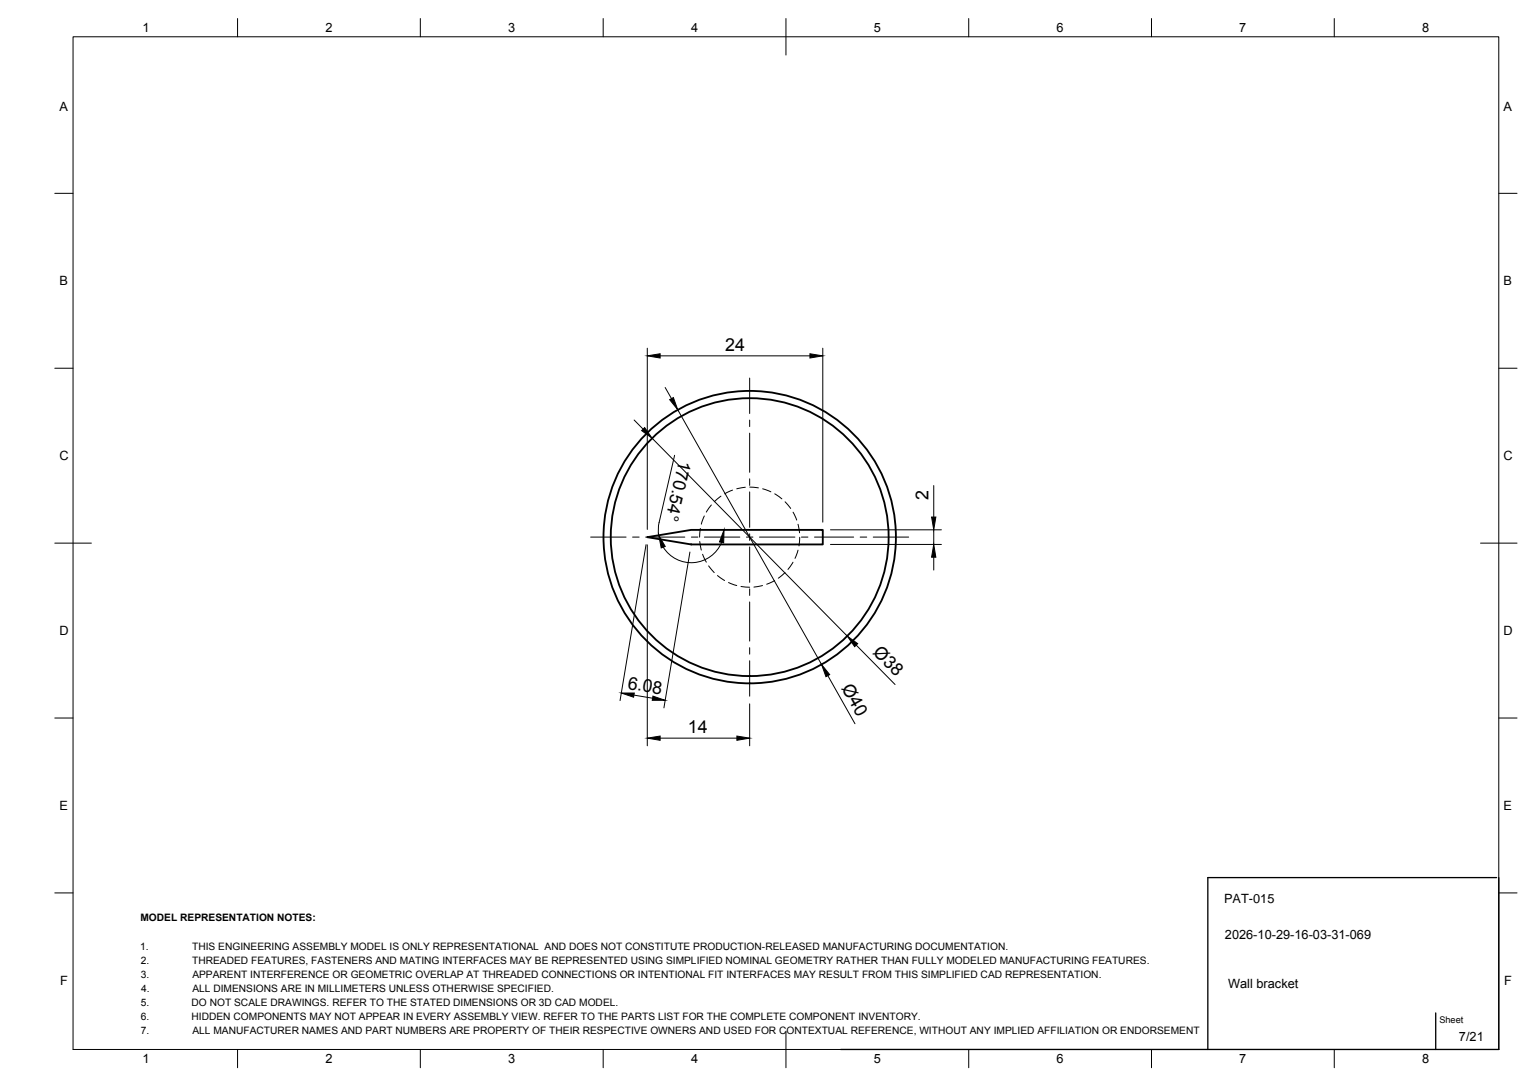
ISO-10303-21;
HEADER;
/* Generated by software containing ST-Developer
 * from STEP Tools, Inc. (www.steptools.com) 
 */

FILE_DESCRIPTION(
/* description */ ('PAT-015'),
/* implementation_level */ '2;1');

FILE_NAME(
/* name */ 'Wall bracket.step',
/* time_stamp */ '2026-10-29T16:03:43-07:00',
/* author */ (''),
/* organization */ (''),
/* preprocessor_version */ 'ST-DEVELOPER v20.2',
/* originating_system */ 'Autodesk Translation Framework v15.17.0.0',
/* authorisation */ '');

FILE_SCHEMA (('AUTOMOTIVE_DESIGN { 1 0 10303 214 3 1 1 }'));
ENDSEC;

DATA;
#10=MECHANICAL_DESIGN_GEOMETRIC_PRESENTATION_REPRESENTATION('',(#236),#10266);
#188=SHAPE_REPRESENTATION_RELATIONSHIP('SRR','None',#10359,#211);
#211=ADVANCED_BREP_SHAPE_REPRESENTATION('',(#261),#10247);
#236=STYLED_ITEM('',(#10526),#261);
#261=MANIFOLD_SOLID_BREP('Body1',#4695);
#346=FACE_BOUND('',#1016,.T.);
#347=FACE_BOUND('',#1017,.T.);
#348=FACE_BOUND('',#1019,.T.);
#349=FACE_BOUND('',#1020,.T.);
#350=FACE_BOUND('',#1024,.T.);
#351=FACE_BOUND('',#1025,.T.);
#352=FACE_BOUND('',#1026,.T.);
#353=FACE_BOUND('',#1027,.T.);
#354=FACE_BOUND('',#1033,.T.);
#355=FACE_BOUND('',#1034,.T.);
#356=FACE_BOUND('',#1035,.T.);
#357=FACE_BOUND('',#1037,.T.);
#358=FACE_BOUND('',#1038,.T.);
#359=FACE_BOUND('',#1039,.T.);
#467=PLANE('',#5185);
#468=PLANE('',#5186);
#469=PLANE('',#5187);
#470=PLANE('',#5188);
#471=PLANE('',#5189);
#472=PLANE('',#5193);
#473=PLANE('',#5194);
#474=PLANE('',#5195);
#475=PLANE('',#5196);
#476=PLANE('',#5197);
#672=FACE_OUTER_BOUND('',#1009,.T.);
#673=FACE_OUTER_BOUND('',#1010,.T.);
#674=FACE_OUTER_BOUND('',#1011,.T.);
#675=FACE_OUTER_BOUND('',#1012,.T.);
#676=FACE_OUTER_BOUND('',#1013,.T.);
#677=FACE_OUTER_BOUND('',#1014,.T.);
#678=FACE_OUTER_BOUND('',#1015,.T.);
#679=FACE_OUTER_BOUND('',#1018,.T.);
#680=FACE_OUTER_BOUND('',#1021,.T.);
#681=FACE_OUTER_BOUND('',#1022,.T.);
#682=FACE_OUTER_BOUND('',#1023,.T.);
#683=FACE_OUTER_BOUND('',#1028,.T.);
#684=FACE_OUTER_BOUND('',#1029,.T.);
#685=FACE_OUTER_BOUND('',#1030,.T.);
#686=FACE_OUTER_BOUND('',#1031,.T.);
#687=FACE_OUTER_BOUND('',#1032,.T.);
#688=FACE_OUTER_BOUND('',#1036,.T.);
#1009=EDGE_LOOP('',(#3553,#3554,#3555,#3556));
#1010=EDGE_LOOP('',(#3557,#3558,#3559,#3560));
#1011=EDGE_LOOP('',(#3561,#3562,#3563,#3564));
#1012=EDGE_LOOP('',(#3565,#3566,#3567,#3568));
#1013=EDGE_LOOP('',(#3569,#3570,#3571,#3572));
#1014=EDGE_LOOP('',(#3573,#3574,#3575,#3576));
#1015=EDGE_LOOP('',(#3577,#3578,#3579,#3580));
#1016=EDGE_LOOP('',(#3581));
#1017=EDGE_LOOP('',(#3582));
#1018=EDGE_LOOP('',(#3583,#3584,#3585,#3586));
#1019=EDGE_LOOP('',(#3587));
#1020=EDGE_LOOP('',(#3588));
#1021=EDGE_LOOP('',(#3589,#3590,#3591,#3592));
#1022=EDGE_LOOP('',(#3593,#3594,#3595,#3596));
#1023=EDGE_LOOP('',(#3597,#3598,#3599,#3600));
#1024=EDGE_LOOP('',(#3601));
#1025=EDGE_LOOP('',(#3602));
#1026=EDGE_LOOP('',(#3603));
#1027=EDGE_LOOP('',(#3604));
#1028=EDGE_LOOP('',(#3605,#3606,#3607,#3608));
#1029=EDGE_LOOP('',(#3609,#3610,#3611,#3612,#3613,#3614,#3615,#3616));
#1030=EDGE_LOOP('',(#3617,#3618,#3619,#3620));
#1031=EDGE_LOOP('',(#3621,#3622,#3623,#3624,#3625,#3626,#3627,#3628));
#1032=EDGE_LOOP('',(#3629,#3630,#3631,#3632));
#1033=EDGE_LOOP('',(#3633));
#1034=EDGE_LOOP('',(#3634));
#1035=EDGE_LOOP('',(#3635));
#1036=EDGE_LOOP('',(#3636,#3637,#3638,#3639));
#1037=EDGE_LOOP('',(#3640));
#1038=EDGE_LOOP('',(#3641));
#1039=EDGE_LOOP('',(#3642));
#1405=LINE('',#8522,#1685);
#1406=LINE('',#8528,#1686);
#1407=LINE('',#8534,#1687);
#1408=LINE('',#8540,#1688);
#1409=LINE('',#8546,#1689);
#1410=LINE('',#8552,#1690);
#1411=LINE('',#8557,#1691);
#1412=LINE('',#8559,#1692);
#1413=LINE('',#8561,#1693);
#1414=LINE('',#8562,#1694);
#1415=LINE('',#8566,#1695);
#1416=LINE('',#8568,#1696);
#1417=LINE('',#8570,#1697);
#1418=LINE('',#8571,#1698);
#1419=LINE('',#8574,#1699);
#1420=LINE('',#8576,#1700);
#1421=LINE('',#8577,#1701);
#1422=LINE('',#8580,#1702);
#1423=LINE('',#8582,#1703);
#1424=LINE('',#8583,#1704);
#1425=LINE('',#8585,#1705);
#1426=LINE('',#8586,#1706);
#1427=LINE('',#8591,#1707);
#1428=LINE('',#8595,#1708);
#1429=LINE('',#8597,#1709);
#1430=LINE('',#8598,#1710);
#1431=LINE('',#8601,#1711);
#1432=LINE('',#8603,#1712);
#1433=LINE('',#8604,#1713);
#1434=LINE('',#8606,#1714);
#1435=LINE('',#8607,#1715);
#1685=VECTOR('',#6036,0.225);
#1686=VECTOR('',#6043,0.225);
#1687=VECTOR('',#6050,0.33);
#1688=VECTOR('',#6057,0.33);
#1689=VECTOR('',#6064,0.33);
#1690=VECTOR('',#6071,0.33);
#1691=VECTOR('',#6076,1.);
#1692=VECTOR('',#6077,1.);
#1693=VECTOR('',#6078,1.);
#1694=VECTOR('',#6079,1.);
#1695=VECTOR('',#6082,1.);
#1696=VECTOR('',#6083,1.);
#1697=VECTOR('',#6084,1.);
#1698=VECTOR('',#6085,1.);
#1699=VECTOR('',#6088,1.);
#1700=VECTOR('',#6089,1.);
#1701=VECTOR('',#6090,1.);
#1702=VECTOR('',#6093,1.);
#1703=VECTOR('',#6094,1.);
#1704=VECTOR('',#6095,1.);
#1705=VECTOR('',#6098,1.);
#1706=VECTOR('',#6099,1.);
#1707=VECTOR('',#6104,3.4);
#1708=VECTOR('',#6109,1.);
#1709=VECTOR('',#6110,1.);
#1710=VECTOR('',#6111,1.);
#1711=VECTOR('',#6114,1.);
#1712=VECTOR('',#6115,1.);
#1713=VECTOR('',#6116,1.);
#1714=VECTOR('',#6119,1.);
#1715=VECTOR('',#6120,1.);
#1959=CIRCLE('',#5168,0.225);
#1960=CIRCLE('',#5169,0.225);
#1961=CIRCLE('',#5171,0.225);
#1962=CIRCLE('',#5172,0.225);
#1963=CIRCLE('',#5174,0.33);
#1964=CIRCLE('',#5175,0.33);
#1965=CIRCLE('',#5177,0.33);
#1966=CIRCLE('',#5178,0.33);
#1967=CIRCLE('',#5180,0.33);
#1968=CIRCLE('',#5181,0.33);
#1969=CIRCLE('',#5183,0.33);
#1970=CIRCLE('',#5184,0.33);
#1971=CIRCLE('',#5191,3.4);
#1972=CIRCLE('',#5192,3.4);
#2265=VERTEX_POINT('',#8519);
#2266=VERTEX_POINT('',#8521);
#2267=VERTEX_POINT('',#8525);
#2268=VERTEX_POINT('',#8527);
#2269=VERTEX_POINT('',#8531);
#2270=VERTEX_POINT('',#8533);
#2271=VERTEX_POINT('',#8537);
#2272=VERTEX_POINT('',#8539);
#2273=VERTEX_POINT('',#8543);
#2274=VERTEX_POINT('',#8545);
#2275=VERTEX_POINT('',#8549);
#2276=VERTEX_POINT('',#8551);
#2277=VERTEX_POINT('',#8555);
#2278=VERTEX_POINT('',#8556);
#2279=VERTEX_POINT('',#8558);
#2280=VERTEX_POINT('',#8560);
#2281=VERTEX_POINT('',#8564);
#2282=VERTEX_POINT('',#8565);
#2283=VERTEX_POINT('',#8567);
#2284=VERTEX_POINT('',#8569);
#2285=VERTEX_POINT('',#8573);
#2286=VERTEX_POINT('',#8575);
#2287=VERTEX_POINT('',#8579);
#2288=VERTEX_POINT('',#8581);
#2289=VERTEX_POINT('',#8588);
#2290=VERTEX_POINT('',#8590);
#2291=VERTEX_POINT('',#8594);
#2292=VERTEX_POINT('',#8596);
#2293=VERTEX_POINT('',#8600);
#2294=VERTEX_POINT('',#8602);
#2732=EDGE_CURVE('',#2265,#2265,#1959,.T.);
#2733=EDGE_CURVE('',#2265,#2266,#1405,.T.);
#2734=EDGE_CURVE('',#2266,#2266,#1960,.T.);
#2735=EDGE_CURVE('',#2267,#2267,#1961,.T.);
#2736=EDGE_CURVE('',#2267,#2268,#1406,.T.);
#2737=EDGE_CURVE('',#2268,#2268,#1962,.T.);
#2738=EDGE_CURVE('',#2269,#2269,#1963,.T.);
#2739=EDGE_CURVE('',#2269,#2270,#1407,.T.);
#2740=EDGE_CURVE('',#2270,#2270,#1964,.T.);
#2741=EDGE_CURVE('',#2271,#2271,#1965,.T.);
#2742=EDGE_CURVE('',#2271,#2272,#1408,.T.);
#2743=EDGE_CURVE('',#2272,#2272,#1966,.T.);
#2744=EDGE_CURVE('',#2273,#2273,#1967,.T.);
#2745=EDGE_CURVE('',#2273,#2274,#1409,.T.);
#2746=EDGE_CURVE('',#2274,#2274,#1968,.T.);
#2747=EDGE_CURVE('',#2275,#2275,#1969,.T.);
#2748=EDGE_CURVE('',#2275,#2276,#1410,.T.);
#2749=EDGE_CURVE('',#2276,#2276,#1970,.T.);
#2750=EDGE_CURVE('',#2277,#2278,#1411,.T.);
#2751=EDGE_CURVE('',#2278,#2279,#1412,.T.);
#2752=EDGE_CURVE('',#2279,#2280,#1413,.T.);
#2753=EDGE_CURVE('',#2280,#2277,#1414,.T.);
#2754=EDGE_CURVE('',#2281,#2282,#1415,.T.);
#2755=EDGE_CURVE('',#2281,#2283,#1416,.T.);
#2756=EDGE_CURVE('',#2283,#2284,#1417,.T.);
#2757=EDGE_CURVE('',#2284,#2282,#1418,.T.);
#2758=EDGE_CURVE('',#2279,#2285,#1419,.T.);
#2759=EDGE_CURVE('',#2286,#2285,#1420,.T.);
#2760=EDGE_CURVE('',#2280,#2286,#1421,.T.);
#2761=EDGE_CURVE('',#2283,#2287,#1422,.T.);
#2762=EDGE_CURVE('',#2288,#2287,#1423,.T.);
#2763=EDGE_CURVE('',#2284,#2288,#1424,.T.);
#2764=EDGE_CURVE('',#2287,#2286,#1425,.T.);
#2765=EDGE_CURVE('',#2285,#2288,#1426,.T.);
#2766=EDGE_CURVE('',#2289,#2289,#1971,.T.);
#2767=EDGE_CURVE('',#2289,#2290,#1427,.T.);
#2768=EDGE_CURVE('',#2290,#2290,#1972,.T.);
#2769=EDGE_CURVE('',#2291,#2277,#1428,.T.);
#2770=EDGE_CURVE('',#2292,#2281,#1429,.T.);
#2771=EDGE_CURVE('',#2291,#2292,#1430,.T.);
#2772=EDGE_CURVE('',#2293,#2291,#1431,.T.);
#2773=EDGE_CURVE('',#2294,#2292,#1432,.T.);
#2774=EDGE_CURVE('',#2293,#2294,#1433,.T.);
#2775=EDGE_CURVE('',#2278,#2293,#1434,.T.);
#2776=EDGE_CURVE('',#2282,#2294,#1435,.T.);
#3553=ORIENTED_EDGE('',*,*,#2732,.F.);
#3554=ORIENTED_EDGE('',*,*,#2733,.T.);
#3555=ORIENTED_EDGE('',*,*,#2734,.F.);
#3556=ORIENTED_EDGE('',*,*,#2733,.F.);
#3557=ORIENTED_EDGE('',*,*,#2735,.F.);
#3558=ORIENTED_EDGE('',*,*,#2736,.T.);
#3559=ORIENTED_EDGE('',*,*,#2737,.F.);
#3560=ORIENTED_EDGE('',*,*,#2736,.F.);
#3561=ORIENTED_EDGE('',*,*,#2738,.F.);
#3562=ORIENTED_EDGE('',*,*,#2739,.T.);
#3563=ORIENTED_EDGE('',*,*,#2740,.F.);
#3564=ORIENTED_EDGE('',*,*,#2739,.F.);
#3565=ORIENTED_EDGE('',*,*,#2741,.F.);
#3566=ORIENTED_EDGE('',*,*,#2742,.T.);
#3567=ORIENTED_EDGE('',*,*,#2743,.F.);
#3568=ORIENTED_EDGE('',*,*,#2742,.F.);
#3569=ORIENTED_EDGE('',*,*,#2744,.F.);
#3570=ORIENTED_EDGE('',*,*,#2745,.T.);
#3571=ORIENTED_EDGE('',*,*,#2746,.F.);
#3572=ORIENTED_EDGE('',*,*,#2745,.F.);
#3573=ORIENTED_EDGE('',*,*,#2747,.F.);
#3574=ORIENTED_EDGE('',*,*,#2748,.T.);
#3575=ORIENTED_EDGE('',*,*,#2749,.F.);
#3576=ORIENTED_EDGE('',*,*,#2748,.F.);
#3577=ORIENTED_EDGE('',*,*,#2750,.T.);
#3578=ORIENTED_EDGE('',*,*,#2751,.T.);
#3579=ORIENTED_EDGE('',*,*,#2752,.T.);
#3580=ORIENTED_EDGE('',*,*,#2753,.T.);
#3581=ORIENTED_EDGE('',*,*,#2738,.T.);
#3582=ORIENTED_EDGE('',*,*,#2744,.T.);
#3583=ORIENTED_EDGE('',*,*,#2754,.F.);
#3584=ORIENTED_EDGE('',*,*,#2755,.T.);
#3585=ORIENTED_EDGE('',*,*,#2756,.T.);
#3586=ORIENTED_EDGE('',*,*,#2757,.T.);
#3587=ORIENTED_EDGE('',*,*,#2741,.T.);
#3588=ORIENTED_EDGE('',*,*,#2747,.T.);
#3589=ORIENTED_EDGE('',*,*,#2752,.F.);
#3590=ORIENTED_EDGE('',*,*,#2758,.T.);
#3591=ORIENTED_EDGE('',*,*,#2759,.F.);
#3592=ORIENTED_EDGE('',*,*,#2760,.F.);
#3593=ORIENTED_EDGE('',*,*,#2756,.F.);
#3594=ORIENTED_EDGE('',*,*,#2761,.T.);
#3595=ORIENTED_EDGE('',*,*,#2762,.F.);
#3596=ORIENTED_EDGE('',*,*,#2763,.F.);
#3597=ORIENTED_EDGE('',*,*,#2762,.T.);
#3598=ORIENTED_EDGE('',*,*,#2764,.T.);
#3599=ORIENTED_EDGE('',*,*,#2759,.T.);
#3600=ORIENTED_EDGE('',*,*,#2765,.T.);
#3601=ORIENTED_EDGE('',*,*,#2740,.T.);
#3602=ORIENTED_EDGE('',*,*,#2743,.T.);
#3603=ORIENTED_EDGE('',*,*,#2746,.T.);
#3604=ORIENTED_EDGE('',*,*,#2749,.T.);
#3605=ORIENTED_EDGE('',*,*,#2766,.F.);
#3606=ORIENTED_EDGE('',*,*,#2767,.T.);
#3607=ORIENTED_EDGE('',*,*,#2768,.F.);
#3608=ORIENTED_EDGE('',*,*,#2767,.F.);
#3609=ORIENTED_EDGE('',*,*,#2769,.T.);
#3610=ORIENTED_EDGE('',*,*,#2753,.F.);
#3611=ORIENTED_EDGE('',*,*,#2760,.T.);
#3612=ORIENTED_EDGE('',*,*,#2764,.F.);
#3613=ORIENTED_EDGE('',*,*,#2761,.F.);
#3614=ORIENTED_EDGE('',*,*,#2755,.F.);
#3615=ORIENTED_EDGE('',*,*,#2770,.F.);
#3616=ORIENTED_EDGE('',*,*,#2771,.F.);
#3617=ORIENTED_EDGE('',*,*,#2772,.T.);
#3618=ORIENTED_EDGE('',*,*,#2771,.T.);
#3619=ORIENTED_EDGE('',*,*,#2773,.F.);
#3620=ORIENTED_EDGE('',*,*,#2774,.F.);
#3621=ORIENTED_EDGE('',*,*,#2775,.T.);
#3622=ORIENTED_EDGE('',*,*,#2774,.T.);
#3623=ORIENTED_EDGE('',*,*,#2776,.F.);
#3624=ORIENTED_EDGE('',*,*,#2757,.F.);
#3625=ORIENTED_EDGE('',*,*,#2763,.T.);
#3626=ORIENTED_EDGE('',*,*,#2765,.F.);
#3627=ORIENTED_EDGE('',*,*,#2758,.F.);
#3628=ORIENTED_EDGE('',*,*,#2751,.F.);
#3629=ORIENTED_EDGE('',*,*,#2776,.T.);
#3630=ORIENTED_EDGE('',*,*,#2773,.T.);
#3631=ORIENTED_EDGE('',*,*,#2770,.T.);
#3632=ORIENTED_EDGE('',*,*,#2754,.T.);
#3633=ORIENTED_EDGE('',*,*,#2734,.T.);
#3634=ORIENTED_EDGE('',*,*,#2737,.T.);
#3635=ORIENTED_EDGE('',*,*,#2768,.T.);
#3636=ORIENTED_EDGE('',*,*,#2775,.F.);
#3637=ORIENTED_EDGE('',*,*,#2750,.F.);
#3638=ORIENTED_EDGE('',*,*,#2769,.F.);
#3639=ORIENTED_EDGE('',*,*,#2772,.F.);
#3640=ORIENTED_EDGE('',*,*,#2732,.T.);
#3641=ORIENTED_EDGE('',*,*,#2735,.T.);
#3642=ORIENTED_EDGE('',*,*,#2766,.T.);
#4344=CYLINDRICAL_SURFACE('',#5167,0.225);
#4345=CYLINDRICAL_SURFACE('',#5170,0.225);
#4346=CYLINDRICAL_SURFACE('',#5173,0.33);
#4347=CYLINDRICAL_SURFACE('',#5176,0.33);
#4348=CYLINDRICAL_SURFACE('',#5179,0.33);
#4349=CYLINDRICAL_SURFACE('',#5182,0.33);
#4350=CYLINDRICAL_SURFACE('',#5190,3.4);
#4507=ADVANCED_FACE('',(#672),#4344,.F.);
#4508=ADVANCED_FACE('',(#673),#4345,.F.);
#4509=ADVANCED_FACE('',(#674),#4346,.F.);
#4510=ADVANCED_FACE('',(#675),#4347,.F.);
#4511=ADVANCED_FACE('',(#676),#4348,.F.);
#4512=ADVANCED_FACE('',(#677),#4349,.F.);
#4513=ADVANCED_FACE('',(#678,#346,#347),#467,.F.);
#4514=ADVANCED_FACE('',(#679,#348,#349),#468,.F.);
#4515=ADVANCED_FACE('',(#680),#469,.T.);
#4516=ADVANCED_FACE('',(#681),#470,.T.);
#4517=ADVANCED_FACE('',(#682,#350,#351,#352,#353),#471,.T.);
#4518=ADVANCED_FACE('',(#683),#4350,.F.);
#4519=ADVANCED_FACE('',(#684),#472,.T.);
#4520=ADVANCED_FACE('',(#685),#473,.T.);
#4521=ADVANCED_FACE('',(#686),#474,.T.);
#4522=ADVANCED_FACE('',(#687,#354,#355,#356),#475,.T.);
#4523=ADVANCED_FACE('',(#688,#357,#358,#359),#476,.F.);
#4695=CLOSED_SHELL('',(#4507,#4508,#4509,#4510,#4511,#4512,#4513,#4514,
#4515,#4516,#4517,#4518,#4519,#4520,#4521,#4522,#4523));
#5166=AXIS2_PLACEMENT_3D('',#8517,#6030,#6031);
#5167=AXIS2_PLACEMENT_3D('',#8518,#6032,#6033);
#5168=AXIS2_PLACEMENT_3D('',#8520,#6034,#6035);
#5169=AXIS2_PLACEMENT_3D('',#8523,#6037,#6038);
#5170=AXIS2_PLACEMENT_3D('',#8524,#6039,#6040);
#5171=AXIS2_PLACEMENT_3D('',#8526,#6041,#6042);
#5172=AXIS2_PLACEMENT_3D('',#8529,#6044,#6045);
#5173=AXIS2_PLACEMENT_3D('',#8530,#6046,#6047);
#5174=AXIS2_PLACEMENT_3D('',#8532,#6048,#6049);
#5175=AXIS2_PLACEMENT_3D('',#8535,#6051,#6052);
#5176=AXIS2_PLACEMENT_3D('',#8536,#6053,#6054);
#5177=AXIS2_PLACEMENT_3D('',#8538,#6055,#6056);
#5178=AXIS2_PLACEMENT_3D('',#8541,#6058,#6059);
#5179=AXIS2_PLACEMENT_3D('',#8542,#6060,#6061);
#5180=AXIS2_PLACEMENT_3D('',#8544,#6062,#6063);
#5181=AXIS2_PLACEMENT_3D('',#8547,#6065,#6066);
#5182=AXIS2_PLACEMENT_3D('',#8548,#6067,#6068);
#5183=AXIS2_PLACEMENT_3D('',#8550,#6069,#6070);
#5184=AXIS2_PLACEMENT_3D('',#8553,#6072,#6073);
#5185=AXIS2_PLACEMENT_3D('',#8554,#6074,#6075);
#5186=AXIS2_PLACEMENT_3D('',#8563,#6080,#6081);
#5187=AXIS2_PLACEMENT_3D('',#8572,#6086,#6087);
#5188=AXIS2_PLACEMENT_3D('',#8578,#6091,#6092);
#5189=AXIS2_PLACEMENT_3D('',#8584,#6096,#6097);
#5190=AXIS2_PLACEMENT_3D('',#8587,#6100,#6101);
#5191=AXIS2_PLACEMENT_3D('',#8589,#6102,#6103);
#5192=AXIS2_PLACEMENT_3D('',#8592,#6105,#6106);
#5193=AXIS2_PLACEMENT_3D('',#8593,#6107,#6108);
#5194=AXIS2_PLACEMENT_3D('',#8599,#6112,#6113);
#5195=AXIS2_PLACEMENT_3D('',#8605,#6117,#6118);
#5196=AXIS2_PLACEMENT_3D('',#8608,#6121,#6122);
#5197=AXIS2_PLACEMENT_3D('',#8609,#6123,#6124);
#6030=DIRECTION('axis',(0.,0.,1.));
#6031=DIRECTION('refdir',(1.,0.,0.));
#6032=DIRECTION('center_axis',(0.,0.,1.));
#6033=DIRECTION('ref_axis',(1.,0.,0.));
#6034=DIRECTION('center_axis',(0.,0.,1.));
#6035=DIRECTION('ref_axis',(1.,0.,0.));
#6036=DIRECTION('',(0.,0.,1.));
#6037=DIRECTION('center_axis',(0.,0.,-1.));
#6038=DIRECTION('ref_axis',(1.,0.,0.));
#6039=DIRECTION('center_axis',(0.,0.,1.));
#6040=DIRECTION('ref_axis',(1.,0.,0.));
#6041=DIRECTION('center_axis',(0.,0.,1.));
#6042=DIRECTION('ref_axis',(1.,0.,0.));
#6043=DIRECTION('',(0.,0.,1.));
#6044=DIRECTION('center_axis',(0.,0.,-1.));
#6045=DIRECTION('ref_axis',(1.,0.,0.));
#6046=DIRECTION('center_axis',(0.,1.,0.));
#6047=DIRECTION('ref_axis',(1.,0.,0.));
#6048=DIRECTION('center_axis',(0.,1.,0.));
#6049=DIRECTION('ref_axis',(1.,0.,0.));
#6050=DIRECTION('',(0.,1.,0.));
#6051=DIRECTION('center_axis',(0.,-1.,0.));
#6052=DIRECTION('ref_axis',(1.,0.,0.));
#6053=DIRECTION('center_axis',(0.,1.,0.));
#6054=DIRECTION('ref_axis',(1.,0.,0.));
#6055=DIRECTION('center_axis',(0.,1.,0.));
#6056=DIRECTION('ref_axis',(1.,0.,0.));
#6057=DIRECTION('',(0.,1.,0.));
#6058=DIRECTION('center_axis',(0.,-1.,0.));
#6059=DIRECTION('ref_axis',(1.,0.,0.));
#6060=DIRECTION('center_axis',(0.,1.,0.));
#6061=DIRECTION('ref_axis',(1.,0.,0.));
#6062=DIRECTION('center_axis',(0.,1.,0.));
#6063=DIRECTION('ref_axis',(1.,0.,0.));
#6064=DIRECTION('',(0.,1.,0.));
#6065=DIRECTION('center_axis',(0.,-1.,0.));
#6066=DIRECTION('ref_axis',(1.,0.,0.));
#6067=DIRECTION('center_axis',(0.,1.,0.));
#6068=DIRECTION('ref_axis',(1.,0.,0.));
#6069=DIRECTION('center_axis',(0.,1.,0.));
#6070=DIRECTION('ref_axis',(1.,0.,0.));
#6071=DIRECTION('',(0.,1.,0.));
#6072=DIRECTION('center_axis',(0.,-1.,0.));
#6073=DIRECTION('ref_axis',(1.,0.,0.));
#6074=DIRECTION('center_axis',(0.,1.,0.));
#6075=DIRECTION('ref_axis',(1.,0.,0.));
#6076=DIRECTION('',(-1.,0.,0.));
#6077=DIRECTION('',(0.,0.,-1.));
#6078=DIRECTION('',(1.,0.,0.));
#6079=DIRECTION('',(0.,0.,1.));
#6080=DIRECTION('center_axis',(0.,1.,0.));
#6081=DIRECTION('ref_axis',(1.,0.,0.));
#6082=DIRECTION('',(-1.,0.,0.));
#6083=DIRECTION('',(0.,0.,1.));
#6084=DIRECTION('',(-1.,0.,0.));
#6085=DIRECTION('',(0.,0.,-1.));
#6086=DIRECTION('center_axis',(0.,0.,-1.));
#6087=DIRECTION('ref_axis',(-1.,0.,0.));
#6088=DIRECTION('',(0.,1.,0.));
#6089=DIRECTION('',(-1.,0.,0.));
#6090=DIRECTION('',(0.,1.,0.));
#6091=DIRECTION('center_axis',(0.,0.,1.));
#6092=DIRECTION('ref_axis',(1.,0.,0.));
#6093=DIRECTION('',(0.,1.,0.));
#6094=DIRECTION('',(1.,0.,0.));
#6095=DIRECTION('',(0.,1.,0.));
#6096=DIRECTION('center_axis',(0.,1.,0.));
#6097=DIRECTION('ref_axis',(0.,0.,1.));
#6098=DIRECTION('',(0.,0.,-1.));
#6099=DIRECTION('',(0.,0.,1.));
#6100=DIRECTION('center_axis',(0.,0.,1.));
#6101=DIRECTION('ref_axis',(1.,0.,0.));
#6102=DIRECTION('center_axis',(0.,0.,1.));
#6103=DIRECTION('ref_axis',(1.,0.,0.));
#6104=DIRECTION('',(0.,0.,1.));
#6105=DIRECTION('center_axis',(0.,0.,-1.));
#6106=DIRECTION('ref_axis',(1.,0.,0.));
#6107=DIRECTION('center_axis',(1.,0.,0.));
#6108=DIRECTION('ref_axis',(0.,1.,0.));
#6109=DIRECTION('',(0.,1.,0.));
#6110=DIRECTION('',(0.,1.,0.));
#6111=DIRECTION('',(0.,0.,1.));
#6112=DIRECTION('center_axis',(0.,-1.,0.));
#6113=DIRECTION('ref_axis',(1.,0.,0.));
#6114=DIRECTION('',(1.,0.,0.));
#6115=DIRECTION('',(1.,0.,0.));
#6116=DIRECTION('',(0.,0.,1.));
#6117=DIRECTION('center_axis',(-1.,0.,0.));
#6118=DIRECTION('ref_axis',(0.,-1.,0.));
#6119=DIRECTION('',(0.,-1.,0.));
#6120=DIRECTION('',(0.,-1.,0.));
#6121=DIRECTION('center_axis',(0.,0.,1.));
#6122=DIRECTION('ref_axis',(1.,0.,0.));
#6123=DIRECTION('center_axis',(0.,0.,1.));
#6124=DIRECTION('ref_axis',(1.,0.,0.));
#8517=CARTESIAN_POINT('',(0.,0.,0.));
#8518=CARTESIAN_POINT('Origin',(-4.,0.,-0.1));
#8519=CARTESIAN_POINT('',(-4.225,-2.75545529808155E-17,0.));
#8520=CARTESIAN_POINT('Origin',(-4.,0.,0.));
#8521=CARTESIAN_POINT('',(-4.225,2.75545529808155E-17,0.6));
#8522=CARTESIAN_POINT('',(-4.225,-2.75545529808155E-17,-0.1));
#8523=CARTESIAN_POINT('Origin',(-4.,0.,0.6));
#8524=CARTESIAN_POINT('Origin',(4.,0.,-0.1));
#8525=CARTESIAN_POINT('',(3.775,-2.75545529808154E-17,0.));
#8526=CARTESIAN_POINT('Origin',(4.,0.,0.));
#8527=CARTESIAN_POINT('',(3.775,2.75545529808154E-17,0.6));
#8528=CARTESIAN_POINT('',(3.775,-2.75545529808154E-17,-0.1));
#8529=CARTESIAN_POINT('Origin',(4.,0.,0.6));
#8530=CARTESIAN_POINT('Origin',(4.,5.4,-3.));
#8531=CARTESIAN_POINT('',(3.67,5.5,-3.));
#8532=CARTESIAN_POINT('Origin',(4.,5.5,-3.));
#8533=CARTESIAN_POINT('',(3.67,6.1,-3.));
#8534=CARTESIAN_POINT('',(3.67,5.4,-3.));
#8535=CARTESIAN_POINT('Origin',(4.,6.1,-3.));
#8536=CARTESIAN_POINT('Origin',(-4.,5.4,4.5));
#8537=CARTESIAN_POINT('',(-4.33,5.5,4.5));
#8538=CARTESIAN_POINT('Origin',(-4.,5.5,4.5));
#8539=CARTESIAN_POINT('',(-4.33,6.1,4.5));
#8540=CARTESIAN_POINT('',(-4.33,5.4,4.5));
#8541=CARTESIAN_POINT('Origin',(-4.,6.1,4.5));
#8542=CARTESIAN_POINT('Origin',(-4.,5.4,-3.));
#8543=CARTESIAN_POINT('',(-4.33,5.5,-3.));
#8544=CARTESIAN_POINT('Origin',(-4.,5.5,-3.));
#8545=CARTESIAN_POINT('',(-4.33,6.1,-3.));
#8546=CARTESIAN_POINT('',(-4.33,5.4,-3.));
#8547=CARTESIAN_POINT('Origin',(-4.,6.1,-3.));
#8548=CARTESIAN_POINT('Origin',(4.,5.4,4.5));
#8549=CARTESIAN_POINT('',(3.67,5.5,4.5));
#8550=CARTESIAN_POINT('Origin',(4.,5.5,4.5));
#8551=CARTESIAN_POINT('',(3.67,6.1,4.5));
#8552=CARTESIAN_POINT('',(3.67,5.4,4.5));
#8553=CARTESIAN_POINT('Origin',(4.,6.1,4.5));
#8554=CARTESIAN_POINT('Origin',(0.,5.5,1.));
#8555=CARTESIAN_POINT('',(5.,5.5,0.));
#8556=CARTESIAN_POINT('',(-5.,5.5,0.));
#8557=CARTESIAN_POINT('',(5.,5.5,0.));
#8558=CARTESIAN_POINT('',(-5.,5.5,-4.));
#8559=CARTESIAN_POINT('',(-5.,5.5,6.));
#8560=CARTESIAN_POINT('',(5.,5.5,-4.));
#8561=CARTESIAN_POINT('',(-5.,5.5,-4.));
#8562=CARTESIAN_POINT('',(5.,5.5,-4.));
#8563=CARTESIAN_POINT('Origin',(0.,5.5,1.));
#8564=CARTESIAN_POINT('',(5.,5.5,0.6));
#8565=CARTESIAN_POINT('',(-5.,5.5,0.6));
#8566=CARTESIAN_POINT('',(5.,5.5,0.6));
#8567=CARTESIAN_POINT('',(5.,5.5,6.));
#8568=CARTESIAN_POINT('',(5.,5.5,-4.));
#8569=CARTESIAN_POINT('',(-5.,5.5,6.));
#8570=CARTESIAN_POINT('',(5.,5.5,6.));
#8571=CARTESIAN_POINT('',(-5.,5.5,6.));
#8572=CARTESIAN_POINT('Origin',(5.,5.5,-4.));
#8573=CARTESIAN_POINT('',(-5.,6.1,-4.));
#8574=CARTESIAN_POINT('',(-5.,5.5,-4.));
#8575=CARTESIAN_POINT('',(5.,6.1,-4.));
#8576=CARTESIAN_POINT('',(-5.,6.1,-4.));
#8577=CARTESIAN_POINT('',(5.,5.5,-4.));
#8578=CARTESIAN_POINT('Origin',(-5.,5.5,6.));
#8579=CARTESIAN_POINT('',(5.,6.1,6.));
#8580=CARTESIAN_POINT('',(5.,5.5,6.));
#8581=CARTESIAN_POINT('',(-5.,6.1,6.));
#8582=CARTESIAN_POINT('',(5.,6.1,6.));
#8583=CARTESIAN_POINT('',(-5.,5.5,6.));
#8584=CARTESIAN_POINT('Origin',(0.,6.1,1.));
#8585=CARTESIAN_POINT('',(5.,6.1,-4.));
#8586=CARTESIAN_POINT('',(-5.,6.1,6.));
#8587=CARTESIAN_POINT('Origin',(0.,0.,-0.1));
#8588=CARTESIAN_POINT('',(-3.4,-4.163799117101E-16,0.));
#8589=CARTESIAN_POINT('Origin',(0.,0.,0.));
#8590=CARTESIAN_POINT('',(-3.4,4.163799117101E-16,0.6));
#8591=CARTESIAN_POINT('',(-3.4,-4.163799117101E-16,-0.1));
#8592=CARTESIAN_POINT('Origin',(0.,0.,0.6));
#8593=CARTESIAN_POINT('Origin',(5.,-4.5,0.));
#8594=CARTESIAN_POINT('',(5.,-4.5,0.));
#8595=CARTESIAN_POINT('',(5.,-4.5,0.));
#8596=CARTESIAN_POINT('',(5.,-4.5,0.6));
#8597=CARTESIAN_POINT('',(5.,-4.5,0.6));
#8598=CARTESIAN_POINT('',(5.,-4.5,0.));
#8599=CARTESIAN_POINT('Origin',(-5.,-4.5,0.));
#8600=CARTESIAN_POINT('',(-5.,-4.5,0.));
#8601=CARTESIAN_POINT('',(-5.,-4.5,0.));
#8602=CARTESIAN_POINT('',(-5.,-4.5,0.6));
#8603=CARTESIAN_POINT('',(-5.,-4.5,0.6));
#8604=CARTESIAN_POINT('',(-5.,-4.5,0.));
#8605=CARTESIAN_POINT('Origin',(-5.,5.5,0.));
#8606=CARTESIAN_POINT('',(-5.,5.5,0.));
#8607=CARTESIAN_POINT('',(-5.,5.5,0.6));
#8608=CARTESIAN_POINT('Origin',(0.,0.5,0.6));
#8609=CARTESIAN_POINT('Origin',(0.,0.5,0.));
#10222=UNCERTAINTY_MEASURE_WITH_UNIT(LENGTH_MEASURE(0.001),#10267,
'DISTANCE_ACCURACY_VALUE',
'Maximum model space distance between geometric entities at asserted c
onnectivities');
#10241=UNCERTAINTY_MEASURE_WITH_UNIT(LENGTH_MEASURE(0.001),#10267,
'DISTANCE_ACCURACY_VALUE',
'Maximum model space distance between geometric entities at asserted c
onnectivities');
#10247=(
GEOMETRIC_REPRESENTATION_CONTEXT(3)
GLOBAL_UNCERTAINTY_ASSIGNED_CONTEXT((#10222))
GLOBAL_UNIT_ASSIGNED_CONTEXT((#10267,#10269,#10270))
REPRESENTATION_CONTEXT('','3D')
);
#10266=(
GEOMETRIC_REPRESENTATION_CONTEXT(3)
GLOBAL_UNCERTAINTY_ASSIGNED_CONTEXT((#10241))
GLOBAL_UNIT_ASSIGNED_CONTEXT((#10267,#10269,#10270))
REPRESENTATION_CONTEXT('','3D')
);
#10267=(
LENGTH_UNIT()
NAMED_UNIT(*)
SI_UNIT(.CENTI.,.METRE.)
);
#10269=(
NAMED_UNIT(*)
PLANE_ANGLE_UNIT()
SI_UNIT($,.RADIAN.)
);
#10270=(
NAMED_UNIT(*)
SI_UNIT($,.STERADIAN.)
SOLID_ANGLE_UNIT()
);
#10276=SHAPE_DEFINITION_REPRESENTATION(#10300,#10359);
#10300=PRODUCT_DEFINITION_SHAPE('',$,#10384);
#10359=SHAPE_REPRESENTATION('',(#5166),#10247);
#10378=PRODUCT_DEFINITION_CONTEXT('part definition',#10452,'design');
#10384=PRODUCT_DEFINITION('Wall bracket','Wall bracket',#10408,
#10378);
#10408=PRODUCT_DEFINITION_FORMATION('',$,#10459);
#10452=APPLICATION_CONTEXT(
'Core Data for Automotive Mechanical Design Process');
#10453=PRODUCT_CONTEXT('part definition',#10452,'mechanical');
#10459=PRODUCT('Wall bracket','Wall bracket',
'Wall bracket',(#10453));
#10520=COLOUR_RGB('Dark Blue',0.08,0.2,0.34);
#10521=FILL_AREA_STYLE_COLOUR('',#10520);
#10522=FILL_AREA_STYLE('',(#10521));
#10523=SURFACE_STYLE_FILL_AREA(#10522);
#10524=SURFACE_SIDE_STYLE('',(#10523));
#10525=SURFACE_STYLE_USAGE(.BOTH.,#10524);
#10526=PRESENTATION_STYLE_ASSIGNMENT((#10525));
ENDSEC;
END-ISO-10303-21;
